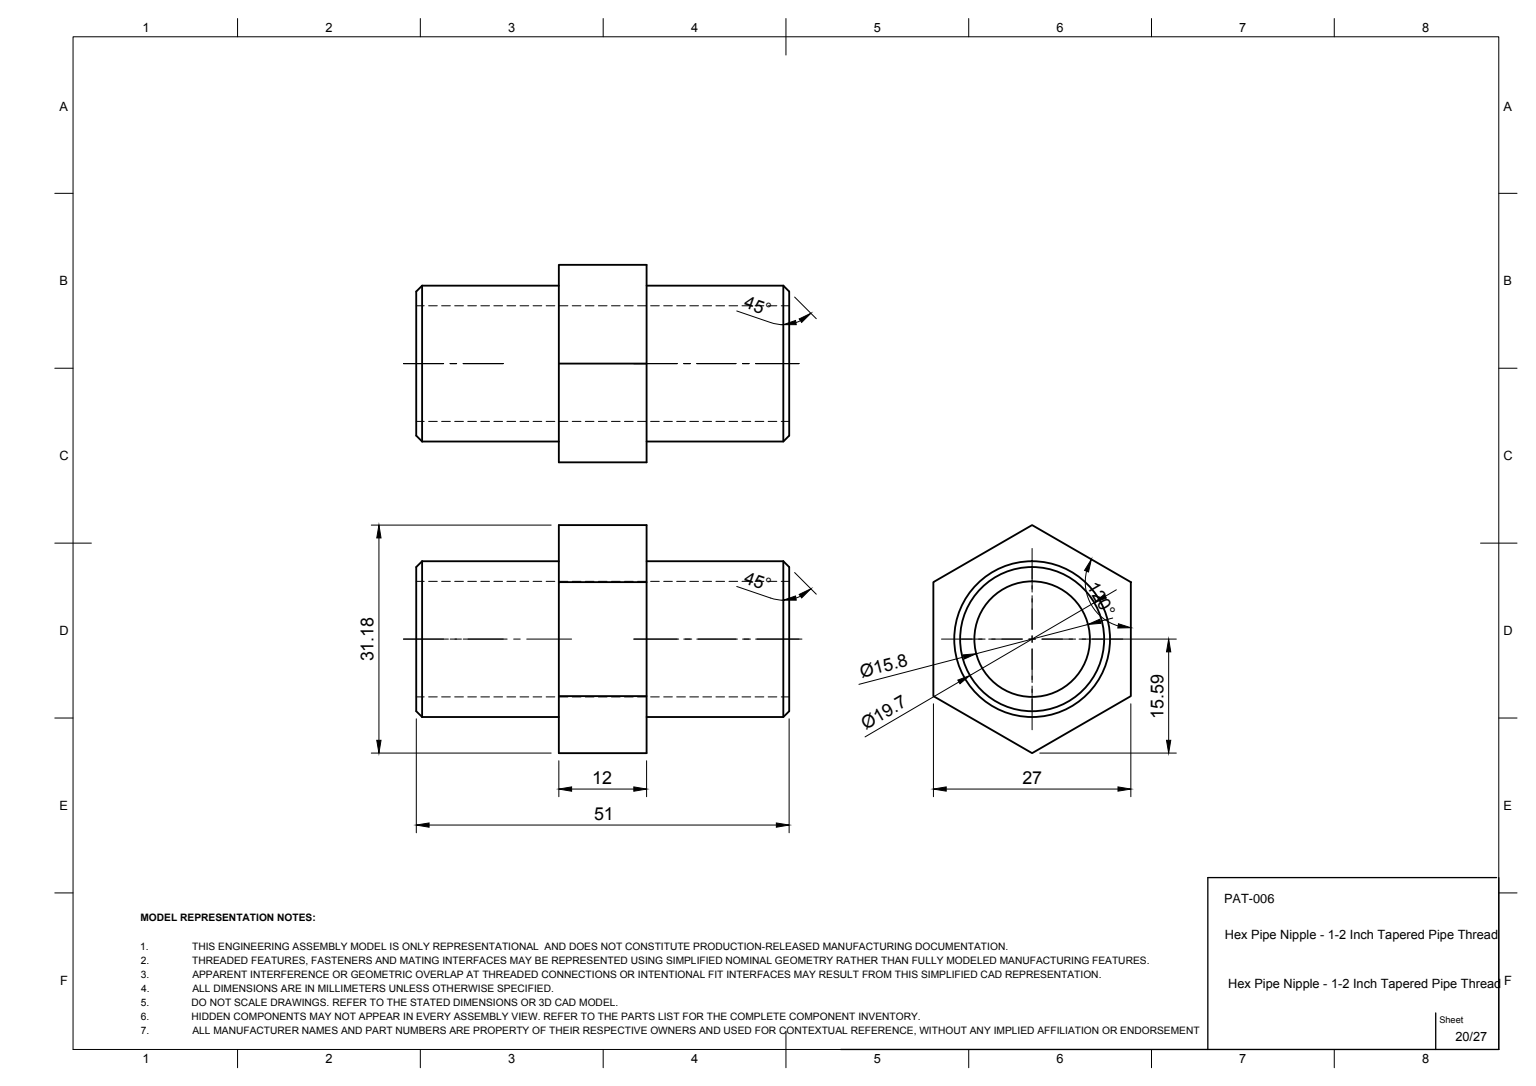
ISO-10303-21;
HEADER;
/* Generated by software containing ST-Developer
 * from STEP Tools, Inc. (www.steptools.com) 
 */

FILE_DESCRIPTION(
/* description */ ('Ball-type isolation valve (generic)'),
/* implementation_level */ '2;1');

FILE_NAME(
/* name */ 'Hex Pipe Nipple - 1-2 Inch Tapered Pipe Thread.step',
/* time_stamp */ '2026-10-27T10:53:05-07:00',
/* author */ (''),
/* organization */ (''),
/* preprocessor_version */ 'ST-DEVELOPER v20.2',
/* originating_system */ 'Autodesk Translation Framework v15.17.0.0',
/* authorisation */ '');

FILE_SCHEMA (('AUTOMOTIVE_DESIGN { 1 0 10303 214 3 1 1 }'));
ENDSEC;

DATA;
#10=MECHANICAL_DESIGN_GEOMETRIC_PRESENTATION_REPRESENTATION('',(#295),#7425);
#209=CONICAL_SURFACE('',#4714,1.025,0.785398163397448);
#210=CONICAL_SURFACE('',#4717,1.025,0.785398163397448);
#243=SHAPE_REPRESENTATION_RELATIONSHIP('SRR','None',#7553,#269);
#269=ADVANCED_BREP_SHAPE_REPRESENTATION('',(#320),#7416);
#295=STYLED_ITEM('',(#7730),#320);
#320=MANIFOLD_SOLID_BREP('Body1',#4101);
#405=FACE_BOUND('',#1055,.T.);
#406=FACE_BOUND('',#1057,.T.);
#407=FACE_BOUND('',#1066,.T.);
#408=FACE_BOUND('',#1071,.T.);
#504=PLANE('',#4699);
#505=PLANE('',#4701);
#506=PLANE('',#4703);
#507=PLANE('',#4704);
#508=PLANE('',#4705);
#509=PLANE('',#4706);
#510=PLANE('',#4707);
#511=PLANE('',#4708);
#512=PLANE('',#4711);
#513=PLANE('',#4719);
#731=FACE_OUTER_BOUND('',#1054,.T.);
#732=FACE_OUTER_BOUND('',#1056,.T.);
#733=FACE_OUTER_BOUND('',#1058,.T.);
#734=FACE_OUTER_BOUND('',#1059,.T.);
#735=FACE_OUTER_BOUND('',#1060,.T.);
#736=FACE_OUTER_BOUND('',#1061,.T.);
#737=FACE_OUTER_BOUND('',#1062,.T.);
#738=FACE_OUTER_BOUND('',#1063,.T.);
#739=FACE_OUTER_BOUND('',#1064,.T.);
#740=FACE_OUTER_BOUND('',#1065,.T.);
#741=FACE_OUTER_BOUND('',#1067,.T.);
#742=FACE_OUTER_BOUND('',#1068,.T.);
#743=FACE_OUTER_BOUND('',#1069,.T.);
#744=FACE_OUTER_BOUND('',#1070,.T.);
#745=FACE_OUTER_BOUND('',#1072,.T.);
#1054=EDGE_LOOP('',(#3369,#3370,#3371,#3372,#3373,#3374));
#1055=EDGE_LOOP('',(#3375));
#1056=EDGE_LOOP('',(#3376,#3377,#3378,#3379,#3380,#3381));
#1057=EDGE_LOOP('',(#3382));
#1058=EDGE_LOOP('',(#3383,#3384,#3385,#3386));
#1059=EDGE_LOOP('',(#3387,#3388,#3389,#3390));
#1060=EDGE_LOOP('',(#3391,#3392,#3393,#3394));
#1061=EDGE_LOOP('',(#3395,#3396,#3397,#3398));
#1062=EDGE_LOOP('',(#3399,#3400,#3401,#3402));
#1063=EDGE_LOOP('',(#3403,#3404,#3405,#3406));
#1064=EDGE_LOOP('',(#3407,#3408,#3409,#3410));
#1065=EDGE_LOOP('',(#3411));
#1066=EDGE_LOOP('',(#3412));
#1067=EDGE_LOOP('',(#3413,#3414,#3415,#3416));
#1068=EDGE_LOOP('',(#3417,#3418,#3419,#3420));
#1069=EDGE_LOOP('',(#3421,#3422,#3423,#3424));
#1070=EDGE_LOOP('',(#3425));
#1071=EDGE_LOOP('',(#3426));
#1072=EDGE_LOOP('',(#3427,#3428,#3429,#3430));
#1322=LINE('',#6894,#1630);
#1323=LINE('',#6896,#1631);
#1324=LINE('',#6898,#1632);
#1325=LINE('',#6900,#1633);
#1326=LINE('',#6902,#1634);
#1327=LINE('',#6903,#1635);
#1328=LINE('',#6909,#1636);
#1329=LINE('',#6911,#1637);
#1330=LINE('',#6913,#1638);
#1331=LINE('',#6915,#1639);
#1332=LINE('',#6917,#1640);
#1333=LINE('',#6918,#1641);
#1334=LINE('',#6922,#1642);
#1335=LINE('',#6923,#1643);
#1336=LINE('',#6925,#1644);
#1337=LINE('',#6927,#1645);
#1338=LINE('',#6929,#1646);
#1339=LINE('',#6931,#1647);
#1340=LINE('',#6935,#1648);
#1341=LINE('',#6943,#1649);
#1342=LINE('',#6947,#1650);
#1343=LINE('',#6951,#1651);
#1344=LINE('',#6956,#1652);
#1630=VECTOR('',#5657,1.);
#1631=VECTOR('',#5658,1.);
#1632=VECTOR('',#5659,1.);
#1633=VECTOR('',#5660,1.);
#1634=VECTOR('',#5661,1.);
#1635=VECTOR('',#5662,1.);
#1636=VECTOR('',#5667,1.);
#1637=VECTOR('',#5668,1.);
#1638=VECTOR('',#5669,1.);
#1639=VECTOR('',#5670,1.);
#1640=VECTOR('',#5671,1.);
#1641=VECTOR('',#5672,1.);
#1642=VECTOR('',#5677,1.);
#1643=VECTOR('',#5678,1.);
#1644=VECTOR('',#5681,1.);
#1645=VECTOR('',#5684,1.);
#1646=VECTOR('',#5687,1.);
#1647=VECTOR('',#5690,1.);
#1648=VECTOR('',#5695,1.065);
#1649=VECTOR('',#5706,1.025);
#1650=VECTOR('',#5711,1.065);
#1651=VECTOR('',#5716,1.025);
#1652=VECTOR('',#5723,0.79);
#1909=CIRCLE('',#4700,1.065);
#1910=CIRCLE('',#4702,1.065);
#1911=CIRCLE('',#4710,1.065);
#1912=CIRCLE('',#4712,0.985);
#1913=CIRCLE('',#4713,0.79);
#1914=CIRCLE('',#4716,1.065);
#1915=CIRCLE('',#4718,0.985);
#1916=CIRCLE('',#4720,0.79);
#2153=VERTEX_POINT('',#6892);
#2154=VERTEX_POINT('',#6893);
#2155=VERTEX_POINT('',#6895);
#2156=VERTEX_POINT('',#6897);
#2157=VERTEX_POINT('',#6899);
#2158=VERTEX_POINT('',#6901);
#2159=VERTEX_POINT('',#6904);
#2160=VERTEX_POINT('',#6907);
#2161=VERTEX_POINT('',#6908);
#2162=VERTEX_POINT('',#6910);
#2163=VERTEX_POINT('',#6912);
#2164=VERTEX_POINT('',#6914);
#2165=VERTEX_POINT('',#6916);
#2166=VERTEX_POINT('',#6919);
#2167=VERTEX_POINT('',#6934);
#2168=VERTEX_POINT('',#6938);
#2169=VERTEX_POINT('',#6940);
#2170=VERTEX_POINT('',#6945);
#2171=VERTEX_POINT('',#6949);
#2172=VERTEX_POINT('',#6953);
#2577=EDGE_CURVE('',#2153,#2154,#1322,.T.);
#2578=EDGE_CURVE('',#2154,#2155,#1323,.T.);
#2579=EDGE_CURVE('',#2155,#2156,#1324,.T.);
#2580=EDGE_CURVE('',#2156,#2157,#1325,.T.);
#2581=EDGE_CURVE('',#2157,#2158,#1326,.T.);
#2582=EDGE_CURVE('',#2158,#2153,#1327,.T.);
#2583=EDGE_CURVE('',#2159,#2159,#1909,.T.);
#2584=EDGE_CURVE('',#2160,#2161,#1328,.T.);
#2585=EDGE_CURVE('',#2161,#2162,#1329,.T.);
#2586=EDGE_CURVE('',#2162,#2163,#1330,.T.);
#2587=EDGE_CURVE('',#2163,#2164,#1331,.T.);
#2588=EDGE_CURVE('',#2164,#2165,#1332,.T.);
#2589=EDGE_CURVE('',#2165,#2160,#1333,.T.);
#2590=EDGE_CURVE('',#2166,#2166,#1910,.T.);
#2591=EDGE_CURVE('',#2160,#2154,#1334,.T.);
#2592=EDGE_CURVE('',#2155,#2165,#1335,.T.);
#2593=EDGE_CURVE('',#2156,#2164,#1336,.T.);
#2594=EDGE_CURVE('',#2157,#2163,#1337,.T.);
#2595=EDGE_CURVE('',#2158,#2162,#1338,.T.);
#2596=EDGE_CURVE('',#2153,#2161,#1339,.T.);
#2597=EDGE_CURVE('',#2166,#2167,#1340,.T.);
#2598=EDGE_CURVE('',#2167,#2167,#1911,.T.);
#2599=EDGE_CURVE('',#2168,#2168,#1912,.T.);
#2600=EDGE_CURVE('',#2169,#2169,#1913,.T.);
#2601=EDGE_CURVE('',#2167,#2168,#1341,.T.);
#2602=EDGE_CURVE('',#2170,#2170,#1914,.T.);
#2603=EDGE_CURVE('',#2170,#2159,#1342,.T.);
#2604=EDGE_CURVE('',#2171,#2171,#1915,.T.);
#2605=EDGE_CURVE('',#2171,#2170,#1343,.T.);
#2606=EDGE_CURVE('',#2172,#2172,#1916,.T.);
#2607=EDGE_CURVE('',#2172,#2169,#1344,.T.);
#3369=ORIENTED_EDGE('',*,*,#2577,.T.);
#3370=ORIENTED_EDGE('',*,*,#2578,.T.);
#3371=ORIENTED_EDGE('',*,*,#2579,.T.);
#3372=ORIENTED_EDGE('',*,*,#2580,.T.);
#3373=ORIENTED_EDGE('',*,*,#2581,.T.);
#3374=ORIENTED_EDGE('',*,*,#2582,.T.);
#3375=ORIENTED_EDGE('',*,*,#2583,.F.);
#3376=ORIENTED_EDGE('',*,*,#2584,.T.);
#3377=ORIENTED_EDGE('',*,*,#2585,.T.);
#3378=ORIENTED_EDGE('',*,*,#2586,.T.);
#3379=ORIENTED_EDGE('',*,*,#2587,.T.);
#3380=ORIENTED_EDGE('',*,*,#2588,.T.);
#3381=ORIENTED_EDGE('',*,*,#2589,.T.);
#3382=ORIENTED_EDGE('',*,*,#2590,.F.);
#3383=ORIENTED_EDGE('',*,*,#2591,.F.);
#3384=ORIENTED_EDGE('',*,*,#2589,.F.);
#3385=ORIENTED_EDGE('',*,*,#2592,.F.);
#3386=ORIENTED_EDGE('',*,*,#2578,.F.);
#3387=ORIENTED_EDGE('',*,*,#2592,.T.);
#3388=ORIENTED_EDGE('',*,*,#2588,.F.);
#3389=ORIENTED_EDGE('',*,*,#2593,.F.);
#3390=ORIENTED_EDGE('',*,*,#2579,.F.);
#3391=ORIENTED_EDGE('',*,*,#2593,.T.);
#3392=ORIENTED_EDGE('',*,*,#2587,.F.);
#3393=ORIENTED_EDGE('',*,*,#2594,.F.);
#3394=ORIENTED_EDGE('',*,*,#2580,.F.);
#3395=ORIENTED_EDGE('',*,*,#2594,.T.);
#3396=ORIENTED_EDGE('',*,*,#2586,.F.);
#3397=ORIENTED_EDGE('',*,*,#2595,.F.);
#3398=ORIENTED_EDGE('',*,*,#2581,.F.);
#3399=ORIENTED_EDGE('',*,*,#2595,.T.);
#3400=ORIENTED_EDGE('',*,*,#2585,.F.);
#3401=ORIENTED_EDGE('',*,*,#2596,.F.);
#3402=ORIENTED_EDGE('',*,*,#2582,.F.);
#3403=ORIENTED_EDGE('',*,*,#2596,.T.);
#3404=ORIENTED_EDGE('',*,*,#2584,.F.);
#3405=ORIENTED_EDGE('',*,*,#2591,.T.);
#3406=ORIENTED_EDGE('',*,*,#2577,.F.);
#3407=ORIENTED_EDGE('',*,*,#2590,.T.);
#3408=ORIENTED_EDGE('',*,*,#2597,.T.);
#3409=ORIENTED_EDGE('',*,*,#2598,.T.);
#3410=ORIENTED_EDGE('',*,*,#2597,.F.);
#3411=ORIENTED_EDGE('',*,*,#2599,.F.);
#3412=ORIENTED_EDGE('',*,*,#2600,.T.);
#3413=ORIENTED_EDGE('',*,*,#2598,.F.);
#3414=ORIENTED_EDGE('',*,*,#2601,.T.);
#3415=ORIENTED_EDGE('',*,*,#2599,.T.);
#3416=ORIENTED_EDGE('',*,*,#2601,.F.);
#3417=ORIENTED_EDGE('',*,*,#2602,.F.);
#3418=ORIENTED_EDGE('',*,*,#2603,.T.);
#3419=ORIENTED_EDGE('',*,*,#2583,.T.);
#3420=ORIENTED_EDGE('',*,*,#2603,.F.);
#3421=ORIENTED_EDGE('',*,*,#2604,.F.);
#3422=ORIENTED_EDGE('',*,*,#2605,.T.);
#3423=ORIENTED_EDGE('',*,*,#2602,.T.);
#3424=ORIENTED_EDGE('',*,*,#2605,.F.);
#3425=ORIENTED_EDGE('',*,*,#2604,.T.);
#3426=ORIENTED_EDGE('',*,*,#2606,.F.);
#3427=ORIENTED_EDGE('',*,*,#2606,.T.);
#3428=ORIENTED_EDGE('',*,*,#2607,.T.);
#3429=ORIENTED_EDGE('',*,*,#2600,.F.);
#3430=ORIENTED_EDGE('',*,*,#2607,.F.);
#3821=CYLINDRICAL_SURFACE('',#4709,1.065);
#3822=CYLINDRICAL_SURFACE('',#4715,1.065);
#3823=CYLINDRICAL_SURFACE('',#4721,0.79);
#3985=ADVANCED_FACE('',(#731,#405),#504,.F.);
#3986=ADVANCED_FACE('',(#732,#406),#505,.T.);
#3987=ADVANCED_FACE('',(#733),#506,.T.);
#3988=ADVANCED_FACE('',(#734),#507,.T.);
#3989=ADVANCED_FACE('',(#735),#508,.T.);
#3990=ADVANCED_FACE('',(#736),#509,.T.);
#3991=ADVANCED_FACE('',(#737),#510,.T.);
#3992=ADVANCED_FACE('',(#738),#511,.T.);
#3993=ADVANCED_FACE('',(#739),#3821,.T.);
#3994=ADVANCED_FACE('',(#740,#407),#512,.T.);
#3995=ADVANCED_FACE('',(#741),#209,.T.);
#3996=ADVANCED_FACE('',(#742),#3822,.T.);
#3997=ADVANCED_FACE('',(#743),#210,.T.);
#3998=ADVANCED_FACE('',(#744,#408),#513,.T.);
#3999=ADVANCED_FACE('',(#745),#3823,.F.);
#4101=CLOSED_SHELL('',(#3985,#3986,#3987,#3988,#3989,#3990,#3991,#3992,
#3993,#3994,#3995,#3996,#3997,#3998,#3999));
#4698=AXIS2_PLACEMENT_3D('',#6890,#5653,#5654);
#4699=AXIS2_PLACEMENT_3D('',#6891,#5655,#5656);
#4700=AXIS2_PLACEMENT_3D('',#6905,#5663,#5664);
#4701=AXIS2_PLACEMENT_3D('',#6906,#5665,#5666);
#4702=AXIS2_PLACEMENT_3D('',#6920,#5673,#5674);
#4703=AXIS2_PLACEMENT_3D('',#6921,#5675,#5676);
#4704=AXIS2_PLACEMENT_3D('',#6924,#5679,#5680);
#4705=AXIS2_PLACEMENT_3D('',#6926,#5682,#5683);
#4706=AXIS2_PLACEMENT_3D('',#6928,#5685,#5686);
#4707=AXIS2_PLACEMENT_3D('',#6930,#5688,#5689);
#4708=AXIS2_PLACEMENT_3D('',#6932,#5691,#5692);
#4709=AXIS2_PLACEMENT_3D('',#6933,#5693,#5694);
#4710=AXIS2_PLACEMENT_3D('',#6936,#5696,#5697);
#4711=AXIS2_PLACEMENT_3D('',#6937,#5698,#5699);
#4712=AXIS2_PLACEMENT_3D('',#6939,#5700,#5701);
#4713=AXIS2_PLACEMENT_3D('',#6941,#5702,#5703);
#4714=AXIS2_PLACEMENT_3D('',#6942,#5704,#5705);
#4715=AXIS2_PLACEMENT_3D('',#6944,#5707,#5708);
#4716=AXIS2_PLACEMENT_3D('',#6946,#5709,#5710);
#4717=AXIS2_PLACEMENT_3D('',#6948,#5712,#5713);
#4718=AXIS2_PLACEMENT_3D('',#6950,#5714,#5715);
#4719=AXIS2_PLACEMENT_3D('',#6952,#5717,#5718);
#4720=AXIS2_PLACEMENT_3D('',#6954,#5719,#5720);
#4721=AXIS2_PLACEMENT_3D('',#6955,#5721,#5722);
#5653=DIRECTION('axis',(0.,0.,1.));
#5654=DIRECTION('refdir',(1.,0.,0.));
#5655=DIRECTION('center_axis',(0.,1.,0.));
#5656=DIRECTION('ref_axis',(1.,0.,0.));
#5657=DIRECTION('',(-0.5,0.,0.866025403784439));
#5658=DIRECTION('',(-1.,0.,-2.84883360945713E-16));
#5659=DIRECTION('',(-0.5,0.,-0.866025403784439));
#5660=DIRECTION('',(0.5,0.,-0.866025403784439));
#5661=DIRECTION('',(1.,0.,0.));
#5662=DIRECTION('',(0.5,0.,0.866025403784439));
#5663=DIRECTION('center_axis',(0.,-1.,0.));
#5664=DIRECTION('ref_axis',(1.,0.,0.));
#5665=DIRECTION('center_axis',(0.,1.,0.));
#5666=DIRECTION('ref_axis',(1.,0.,0.));
#5667=DIRECTION('',(0.5,0.,-0.866025403784439));
#5668=DIRECTION('',(-0.5,0.,-0.866025403784439));
#5669=DIRECTION('',(-1.,0.,0.));
#5670=DIRECTION('',(-0.5,0.,0.866025403784439));
#5671=DIRECTION('',(0.5,0.,0.866025403784439));
#5672=DIRECTION('',(1.,0.,2.84883360945713E-16));
#5673=DIRECTION('center_axis',(0.,1.,0.));
#5674=DIRECTION('ref_axis',(1.,0.,0.));
#5675=DIRECTION('center_axis',(-2.84883360945713E-16,0.,1.));
#5676=DIRECTION('ref_axis',(1.,0.,2.84883360945713E-16));
#5677=DIRECTION('',(0.,-1.,0.));
#5678=DIRECTION('',(0.,1.,0.));
#5679=DIRECTION('center_axis',(-0.866025403784439,0.,0.5));
#5680=DIRECTION('ref_axis',(0.5,0.,0.866025403784439));
#5681=DIRECTION('',(0.,1.,0.));
#5682=DIRECTION('center_axis',(-0.866025403784439,0.,-0.5));
#5683=DIRECTION('ref_axis',(-0.5,0.,0.866025403784439));
#5684=DIRECTION('',(0.,1.,0.));
#5685=DIRECTION('center_axis',(0.,0.,-1.));
#5686=DIRECTION('ref_axis',(-1.,0.,0.));
#5687=DIRECTION('',(0.,1.,0.));
#5688=DIRECTION('center_axis',(0.866025403784439,0.,-0.5));
#5689=DIRECTION('ref_axis',(-0.5,0.,-0.866025403784439));
#5690=DIRECTION('',(0.,1.,0.));
#5691=DIRECTION('center_axis',(0.866025403784439,0.,0.5));
#5692=DIRECTION('ref_axis',(0.5,0.,-0.866025403784439));
#5693=DIRECTION('center_axis',(0.,-1.,0.));
#5694=DIRECTION('ref_axis',(1.,0.,0.));
#5695=DIRECTION('',(0.,1.,0.));
#5696=DIRECTION('center_axis',(0.,-1.,0.));
#5697=DIRECTION('ref_axis',(1.,0.,0.));
#5698=DIRECTION('center_axis',(0.,1.,0.));
#5699=DIRECTION('ref_axis',(0.,0.,1.));
#5700=DIRECTION('center_axis',(0.,-1.,0.));
#5701=DIRECTION('ref_axis',(1.,0.,0.));
#5702=DIRECTION('center_axis',(0.,-1.,0.));
#5703=DIRECTION('ref_axis',(1.,0.,0.));
#5704=DIRECTION('center_axis',(0.,-1.,0.));
#5705=DIRECTION('ref_axis',(1.,0.,0.));
#5706=DIRECTION('',(0.707106781186547,0.707106781186548,8.65956056235493E-17));
#5707=DIRECTION('center_axis',(0.,-1.,0.));
#5708=DIRECTION('ref_axis',(1.,0.,0.));
#5709=DIRECTION('center_axis',(0.,-1.,0.));
#5710=DIRECTION('ref_axis',(1.,0.,0.));
#5711=DIRECTION('',(0.,1.,0.));
#5712=DIRECTION('center_axis',(0.,1.,0.));
#5713=DIRECTION('ref_axis',(1.,0.,0.));
#5714=DIRECTION('center_axis',(0.,-1.,0.));
#5715=DIRECTION('ref_axis',(1.,0.,0.));
#5716=DIRECTION('',(-0.707106781186547,0.707106781186548,-8.65956056235493E-17));
#5717=DIRECTION('center_axis',(0.,-1.,0.));
#5718=DIRECTION('ref_axis',(0.,0.,-1.));
#5719=DIRECTION('center_axis',(0.,-1.,0.));
#5720=DIRECTION('ref_axis',(1.,0.,0.));
#5721=DIRECTION('center_axis',(0.,-1.,0.));
#5722=DIRECTION('ref_axis',(1.,0.,0.));
#5723=DIRECTION('',(0.,1.,0.));
#6890=CARTESIAN_POINT('',(0.,0.,0.));
#6891=CARTESIAN_POINT('Origin',(0.,-0.6,0.));
#6892=CARTESIAN_POINT('',(1.55884572681199,-0.6,0.));
#6893=CARTESIAN_POINT('',(0.779422863405995,-0.6,1.35));
#6894=CARTESIAN_POINT('',(0.779422863405995,-0.6,1.35));
#6895=CARTESIAN_POINT('',(-0.779422863405996,-0.6,1.35));
#6896=CARTESIAN_POINT('',(-0.779422863405996,-0.6,1.35));
#6897=CARTESIAN_POINT('',(-1.55884572681199,-0.6,-1.90903542970483E-16));
#6898=CARTESIAN_POINT('',(-1.55884572681199,-0.6,-1.90903542970483E-16));
#6899=CARTESIAN_POINT('',(-0.779422863405995,-0.6,-1.35));
#6900=CARTESIAN_POINT('',(-0.779422863405995,-0.6,-1.35));
#6901=CARTESIAN_POINT('',(0.779422863405995,-0.6,-1.35));
#6902=CARTESIAN_POINT('',(0.779422863405995,-0.6,-1.35));
#6903=CARTESIAN_POINT('',(1.55884572681199,-0.6,0.));
#6904=CARTESIAN_POINT('',(-1.065,-0.6,-1.30424884109193E-16));
#6905=CARTESIAN_POINT('Origin',(0.,-0.6,0.));
#6906=CARTESIAN_POINT('Origin',(0.,0.6,0.));
#6907=CARTESIAN_POINT('',(0.779422863405995,0.6,1.35));
#6908=CARTESIAN_POINT('',(1.55884572681199,0.6,0.));
#6909=CARTESIAN_POINT('',(0.779422863405995,0.6,1.35));
#6910=CARTESIAN_POINT('',(0.779422863405995,0.6,-1.35));
#6911=CARTESIAN_POINT('',(1.55884572681199,0.6,0.));
#6912=CARTESIAN_POINT('',(-0.779422863405995,0.6,-1.35));
#6913=CARTESIAN_POINT('',(0.779422863405995,0.6,-1.35));
#6914=CARTESIAN_POINT('',(-1.55884572681199,0.6,-1.90903542970483E-16));
#6915=CARTESIAN_POINT('',(-0.779422863405995,0.6,-1.35));
#6916=CARTESIAN_POINT('',(-0.779422863405996,0.6,1.35));
#6917=CARTESIAN_POINT('',(-1.55884572681199,0.6,-1.90903542970483E-16));
#6918=CARTESIAN_POINT('',(-0.779422863405996,0.6,1.35));
#6919=CARTESIAN_POINT('',(-1.065,0.6,1.30424884109193E-16));
#6920=CARTESIAN_POINT('Origin',(0.,0.6,0.));
#6921=CARTESIAN_POINT('Origin',(-0.779422863405996,0.,1.35));
#6922=CARTESIAN_POINT('',(0.779422863405995,0.,1.35));
#6923=CARTESIAN_POINT('',(-0.779422863405996,0.,1.35));
#6924=CARTESIAN_POINT('Origin',(-1.55884572681199,0.,-1.90903542970483E-16));
#6925=CARTESIAN_POINT('',(-1.55884572681199,0.,-1.90903542970483E-16));
#6926=CARTESIAN_POINT('Origin',(-0.779422863405995,0.,-1.35));
#6927=CARTESIAN_POINT('',(-0.779422863405995,0.,-1.35));
#6928=CARTESIAN_POINT('Origin',(0.779422863405995,0.,-1.35));
#6929=CARTESIAN_POINT('',(0.779422863405995,0.,-1.35));
#6930=CARTESIAN_POINT('Origin',(1.55884572681199,0.,0.));
#6931=CARTESIAN_POINT('',(1.55884572681199,0.,0.));
#6932=CARTESIAN_POINT('Origin',(0.779422863405995,0.,1.35));
#6933=CARTESIAN_POINT('Origin',(0.,0.,0.));
#6934=CARTESIAN_POINT('',(-1.065,2.47,-1.30424884109193E-16));
#6935=CARTESIAN_POINT('',(-1.065,0.,-1.30424884109193E-16));
#6936=CARTESIAN_POINT('Origin',(0.,2.47,0.));
#6937=CARTESIAN_POINT('Origin',(0.985,2.55,0.));
#6938=CARTESIAN_POINT('',(-0.985,2.55,-1.20627709716014E-16));
#6939=CARTESIAN_POINT('Origin',(0.,2.55,0.));
#6940=CARTESIAN_POINT('',(-0.79,2.55,-9.67470971326409E-17));
#6941=CARTESIAN_POINT('Origin',(0.,2.55,0.));
#6942=CARTESIAN_POINT('Origin',(0.,2.51,0.));
#6943=CARTESIAN_POINT('',(-1.025,2.51,-1.25526296912604E-16));
#6944=CARTESIAN_POINT('Origin',(0.,0.,0.));
#6945=CARTESIAN_POINT('',(-1.065,-2.47,-1.30424884109193E-16));
#6946=CARTESIAN_POINT('Origin',(0.,-2.47,0.));
#6947=CARTESIAN_POINT('',(-1.065,0.,-1.30424884109193E-16));
#6948=CARTESIAN_POINT('Origin',(0.,-2.51,0.));
#6949=CARTESIAN_POINT('',(-0.985,-2.55,-1.20627709716014E-16));
#6950=CARTESIAN_POINT('Origin',(0.,-2.55,0.));
#6951=CARTESIAN_POINT('',(-1.025,-2.51,-1.25526296912604E-16));
#6952=CARTESIAN_POINT('Origin',(0.79,-2.55,0.));
#6953=CARTESIAN_POINT('',(-0.79,-2.55,-9.67470971326409E-17));
#6954=CARTESIAN_POINT('Origin',(0.,-2.55,0.));
#6955=CARTESIAN_POINT('Origin',(0.,0.,0.));
#6956=CARTESIAN_POINT('',(-0.79,0.,-9.67470971326409E-17));
#7386=UNCERTAINTY_MEASURE_WITH_UNIT(LENGTH_MEASURE(0.001),#7426,
'DISTANCE_ACCURACY_VALUE',
'Maximum model space distance between geometric entities at asserted c
onnectivities');
#7395=UNCERTAINTY_MEASURE_WITH_UNIT(LENGTH_MEASURE(0.001),#7426,
'DISTANCE_ACCURACY_VALUE',
'Maximum model space distance between geometric entities at asserted c
onnectivities');
#7416=(
GEOMETRIC_REPRESENTATION_CONTEXT(3)
GLOBAL_UNCERTAINTY_ASSIGNED_CONTEXT((#7386))
GLOBAL_UNIT_ASSIGNED_CONTEXT((#7426,#7428,#7429))
REPRESENTATION_CONTEXT('','3D')
);
#7425=(
GEOMETRIC_REPRESENTATION_CONTEXT(3)
GLOBAL_UNCERTAINTY_ASSIGNED_CONTEXT((#7395))
GLOBAL_UNIT_ASSIGNED_CONTEXT((#7426,#7428,#7429))
REPRESENTATION_CONTEXT('','3D')
);
#7426=(
LENGTH_UNIT()
NAMED_UNIT(*)
SI_UNIT(.CENTI.,.METRE.)
);
#7428=(
NAMED_UNIT(*)
PLANE_ANGLE_UNIT()
SI_UNIT($,.RADIAN.)
);
#7429=(
NAMED_UNIT(*)
SI_UNIT($,.STERADIAN.)
SOLID_ANGLE_UNIT()
);
#7450=SHAPE_DEFINITION_REPRESENTATION(#7479,#7553);
#7479=PRODUCT_DEFINITION_SHAPE('',$,#7583);
#7553=SHAPE_REPRESENTATION('',(#4698),#7416);
#7562=PRODUCT_DEFINITION_CONTEXT('part definition',#7651,'design');
#7583=PRODUCT_DEFINITION(
'Hex Pipe Nipple - 1-2 Inch Tapered Pipe Thread',
'Hex Pipe Nipple - 1-2 Inch Tapered Pipe Thread',#7612,#7562);
#7612=PRODUCT_DEFINITION_FORMATION('',$,#7673);
#7651=APPLICATION_CONTEXT(
'Core Data for Automotive Mechanical Design Process');
#7652=PRODUCT_CONTEXT('part definition',#7651,'mechanical');
#7673=PRODUCT('Hex Pipe Nipple - 1-2 Inch Tapered Pipe Thread',
'Hex Pipe Nipple - 1-2 Inch Tapered Pipe Thread',
'Hex Pipe Nipple - 1-2 Inch Tapered Pipe Thread',(#7652));
#7724=COLOUR_RGB('Light Blue',0.38,0.62,0.78);
#7725=FILL_AREA_STYLE_COLOUR('',#7724);
#7726=FILL_AREA_STYLE('',(#7725));
#7727=SURFACE_STYLE_FILL_AREA(#7726);
#7728=SURFACE_SIDE_STYLE('',(#7727));
#7729=SURFACE_STYLE_USAGE(.BOTH.,#7728);
#7730=PRESENTATION_STYLE_ASSIGNMENT((#7729));
ENDSEC;
END-ISO-10303-21;
